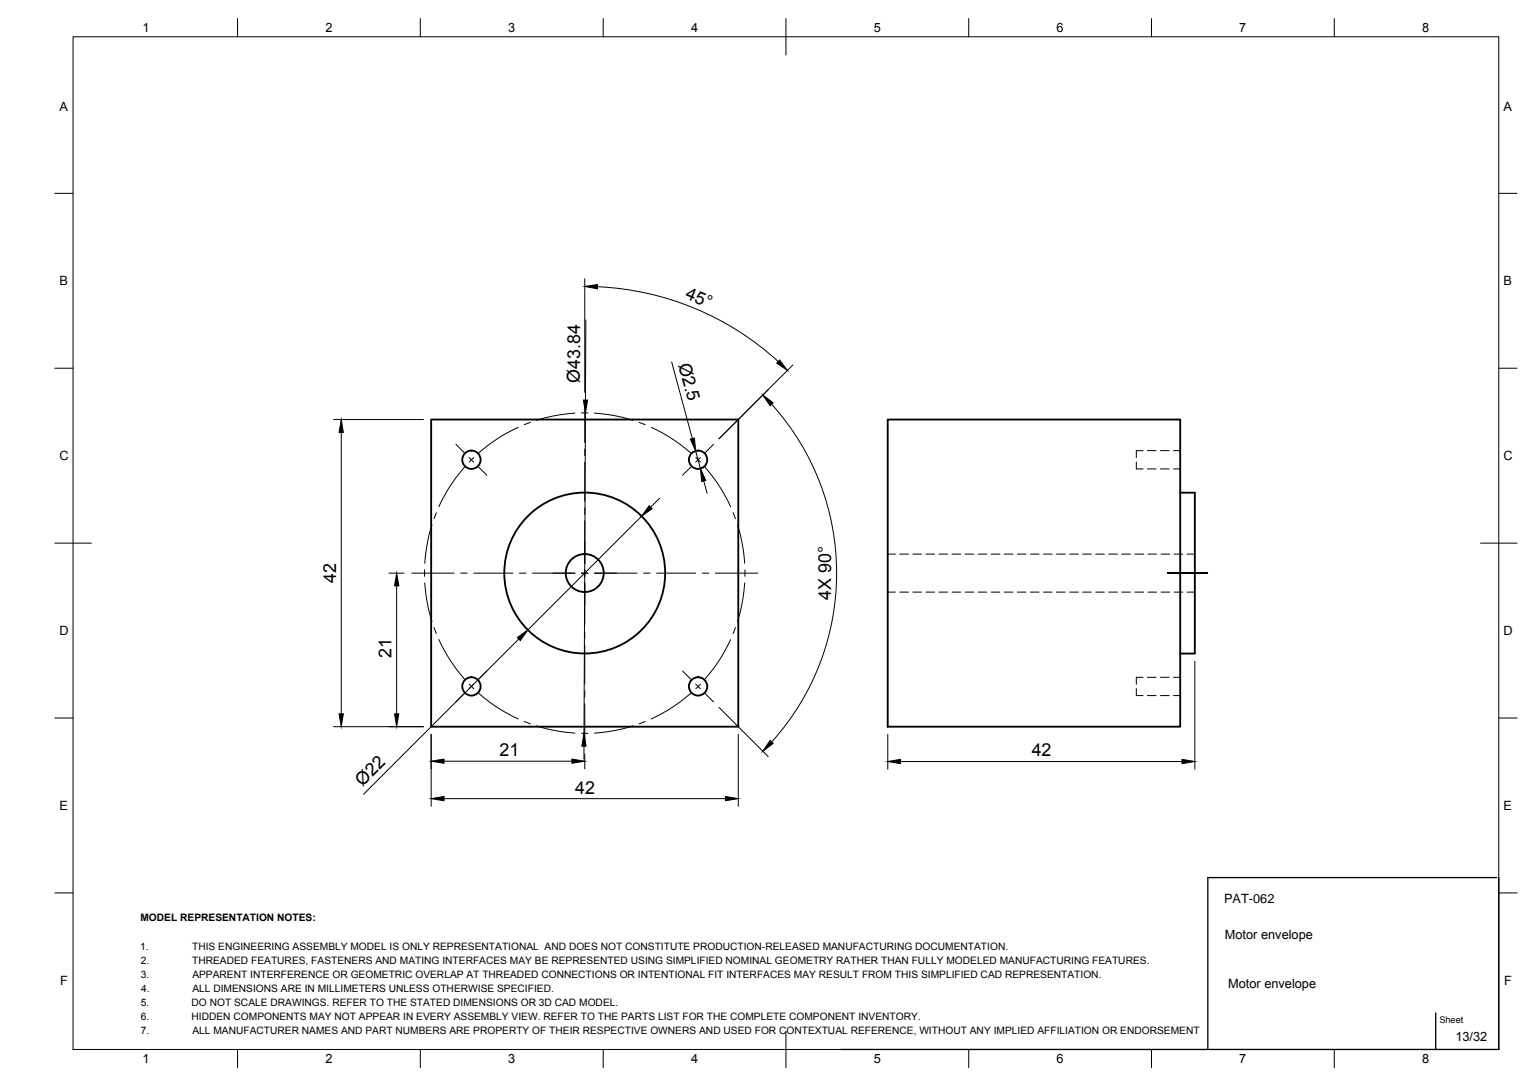
ISO-10303-21;
HEADER;
/* Generated by software containing ST-Developer
 * from STEP Tools, Inc. (www.steptools.com) 
 */

FILE_DESCRIPTION(
/* description */ ('Jaw-coupled motor to shaft test stand'),
/* implementation_level */ '2;1');

FILE_NAME(
/* name */ 'Motor envelope.step',
/* time_stamp */ '2026-10-27T10:46:06-07:00',
/* author */ (''),
/* organization */ (''),
/* preprocessor_version */ 'ST-DEVELOPER v20.2',
/* originating_system */ 'Autodesk Translation Framework v15.17.0.0',
/* authorisation */ '');

FILE_SCHEMA (('AUTOMOTIVE_DESIGN { 1 0 10303 214 3 1 1 }'));
ENDSEC;

DATA;
#10=MECHANICAL_DESIGN_GEOMETRIC_PRESENTATION_REPRESENTATION('',(#348),#19361);
#284=SHAPE_REPRESENTATION_RELATIONSHIP('SRR','None',#19498,#316);
#316=ADVANCED_BREP_SHAPE_REPRESENTATION('',(#381),#19334);
#348=STYLED_ITEM('',(#19739),#381);
#381=MANIFOLD_SOLID_BREP('Body1',#10992);
#437=FACE_BOUND('',#1741,.T.);
#438=FACE_BOUND('',#1744,.T.);
#439=FACE_BOUND('',#1745,.T.);
#440=FACE_BOUND('',#1746,.T.);
#441=FACE_BOUND('',#1747,.T.);
#442=FACE_BOUND('',#1748,.T.);
#443=FACE_BOUND('',#1751,.T.);
#550=PLANE('',#11484);
#551=PLANE('',#11488);
#552=PLANE('',#11492);
#553=PLANE('',#11496);
#554=PLANE('',#11500);
#555=PLANE('',#11504);
#556=PLANE('',#11505);
#557=PLANE('',#11506);
#558=PLANE('',#11507);
#559=PLANE('',#11508);
#560=PLANE('',#11509);
#1077=FACE_OUTER_BOUND('',#1731,.T.);
#1078=FACE_OUTER_BOUND('',#1732,.T.);
#1079=FACE_OUTER_BOUND('',#1733,.T.);
#1080=FACE_OUTER_BOUND('',#1734,.T.);
#1081=FACE_OUTER_BOUND('',#1735,.T.);
#1082=FACE_OUTER_BOUND('',#1736,.T.);
#1083=FACE_OUTER_BOUND('',#1737,.T.);
#1084=FACE_OUTER_BOUND('',#1738,.T.);
#1085=FACE_OUTER_BOUND('',#1739,.T.);
#1086=FACE_OUTER_BOUND('',#1740,.T.);
#1087=FACE_OUTER_BOUND('',#1742,.T.);
#1088=FACE_OUTER_BOUND('',#1743,.T.);
#1089=FACE_OUTER_BOUND('',#1749,.T.);
#1090=FACE_OUTER_BOUND('',#1750,.T.);
#1091=FACE_OUTER_BOUND('',#1752,.T.);
#1092=FACE_OUTER_BOUND('',#1753,.T.);
#1093=FACE_OUTER_BOUND('',#1754,.T.);
#1731=EDGE_LOOP('',(#7580,#7581,#7582,#7583));
#1732=EDGE_LOOP('',(#7584));
#1733=EDGE_LOOP('',(#7585,#7586,#7587,#7588));
#1734=EDGE_LOOP('',(#7589));
#1735=EDGE_LOOP('',(#7590,#7591,#7592,#7593));
#1736=EDGE_LOOP('',(#7594));
#1737=EDGE_LOOP('',(#7595,#7596,#7597,#7598));
#1738=EDGE_LOOP('',(#7599));
#1739=EDGE_LOOP('',(#7600,#7601,#7602,#7603));
#1740=EDGE_LOOP('',(#7604));
#1741=EDGE_LOOP('',(#7605));
#1742=EDGE_LOOP('',(#7606,#7607,#7608,#7609));
#1743=EDGE_LOOP('',(#7610,#7611,#7612,#7613));
#1744=EDGE_LOOP('',(#7614));
#1745=EDGE_LOOP('',(#7615));
#1746=EDGE_LOOP('',(#7616));
#1747=EDGE_LOOP('',(#7617));
#1748=EDGE_LOOP('',(#7618));
#1749=EDGE_LOOP('',(#7619,#7620,#7621,#7622));
#1750=EDGE_LOOP('',(#7623,#7624,#7625,#7626));
#1751=EDGE_LOOP('',(#7627));
#1752=EDGE_LOOP('',(#7628,#7629,#7630,#7631));
#1753=EDGE_LOOP('',(#7632,#7633,#7634,#7635));
#1754=EDGE_LOOP('',(#7636,#7637,#7638,#7639));
#2450=LINE('',#15692,#3603);
#2451=LINE('',#15699,#3604);
#2452=LINE('',#15706,#3605);
#2453=LINE('',#15713,#3606);
#2454=LINE('',#15720,#3607);
#2455=LINE('',#15728,#3608);
#2456=LINE('',#15732,#3609);
#2457=LINE('',#15734,#3610);
#2458=LINE('',#15736,#3611);
#2459=LINE('',#15737,#3612);
#2460=LINE('',#15740,#3613);
#2461=LINE('',#15742,#3614);
#2462=LINE('',#15743,#3615);
#2463=LINE('',#15746,#3616);
#2464=LINE('',#15748,#3617);
#2465=LINE('',#15749,#3618);
#2466=LINE('',#15751,#3619);
#2467=LINE('',#15752,#3620);
#3603=VECTOR('',#12635,0.125);
#3604=VECTOR('',#12644,0.125);
#3605=VECTOR('',#12653,0.125);
#3606=VECTOR('',#12662,0.125);
#3607=VECTOR('',#12671,1.1);
#3608=VECTOR('',#12682,0.26);
#3609=VECTOR('',#12685,1.);
#3610=VECTOR('',#12686,1.);
#3611=VECTOR('',#12687,1.);
#3612=VECTOR('',#12688,1.);
#3613=VECTOR('',#12691,1.);
#3614=VECTOR('',#12692,1.);
#3615=VECTOR('',#12693,1.);
#3616=VECTOR('',#12696,1.);
#3617=VECTOR('',#12697,1.);
#3618=VECTOR('',#12698,1.);
#3619=VECTOR('',#12701,1.);
#3620=VECTOR('',#12702,1.);
#4723=CIRCLE('',#11482,0.125);
#4724=CIRCLE('',#11483,0.125);
#4725=CIRCLE('',#11486,0.125);
#4726=CIRCLE('',#11487,0.125);
#4727=CIRCLE('',#11490,0.125);
#4728=CIRCLE('',#11491,0.125);
#4729=CIRCLE('',#11494,0.125);
#4730=CIRCLE('',#11495,0.125);
#4731=CIRCLE('',#11498,1.1);
#4732=CIRCLE('',#11499,1.1);
#4733=CIRCLE('',#11501,0.26);
#4734=CIRCLE('',#11503,0.26);
#5021=VERTEX_POINT('',#15689);
#5022=VERTEX_POINT('',#15691);
#5023=VERTEX_POINT('',#15696);
#5024=VERTEX_POINT('',#15698);
#5025=VERTEX_POINT('',#15703);
#5026=VERTEX_POINT('',#15705);
#5027=VERTEX_POINT('',#15710);
#5028=VERTEX_POINT('',#15712);
#5029=VERTEX_POINT('',#15717);
#5030=VERTEX_POINT('',#15719);
#5031=VERTEX_POINT('',#15723);
#5032=VERTEX_POINT('',#15726);
#5033=VERTEX_POINT('',#15730);
#5034=VERTEX_POINT('',#15731);
#5035=VERTEX_POINT('',#15733);
#5036=VERTEX_POINT('',#15735);
#5037=VERTEX_POINT('',#15739);
#5038=VERTEX_POINT('',#15741);
#5039=VERTEX_POINT('',#15745);
#5040=VERTEX_POINT('',#15747);
#6001=EDGE_CURVE('',#5021,#5021,#4723,.T.);
#6002=EDGE_CURVE('',#5021,#5022,#2450,.T.);
#6003=EDGE_CURVE('',#5022,#5022,#4724,.T.);
#6004=EDGE_CURVE('',#5023,#5023,#4725,.T.);
#6005=EDGE_CURVE('',#5023,#5024,#2451,.T.);
#6006=EDGE_CURVE('',#5024,#5024,#4726,.T.);
#6007=EDGE_CURVE('',#5025,#5025,#4727,.T.);
#6008=EDGE_CURVE('',#5025,#5026,#2452,.T.);
#6009=EDGE_CURVE('',#5026,#5026,#4728,.T.);
#6010=EDGE_CURVE('',#5027,#5027,#4729,.T.);
#6011=EDGE_CURVE('',#5027,#5028,#2453,.T.);
#6012=EDGE_CURVE('',#5028,#5028,#4730,.T.);
#6013=EDGE_CURVE('',#5029,#5029,#4731,.T.);
#6014=EDGE_CURVE('',#5029,#5030,#2454,.T.);
#6015=EDGE_CURVE('',#5030,#5030,#4732,.T.);
#6016=EDGE_CURVE('',#5031,#5031,#4733,.T.);
#6017=EDGE_CURVE('',#5032,#5032,#4734,.T.);
#6018=EDGE_CURVE('',#5032,#5031,#2455,.T.);
#6019=EDGE_CURVE('',#5033,#5034,#2456,.T.);
#6020=EDGE_CURVE('',#5034,#5035,#2457,.T.);
#6021=EDGE_CURVE('',#5036,#5035,#2458,.T.);
#6022=EDGE_CURVE('',#5033,#5036,#2459,.T.);
#6023=EDGE_CURVE('',#5037,#5033,#2460,.T.);
#6024=EDGE_CURVE('',#5038,#5036,#2461,.T.);
#6025=EDGE_CURVE('',#5037,#5038,#2462,.T.);
#6026=EDGE_CURVE('',#5039,#5037,#2463,.T.);
#6027=EDGE_CURVE('',#5040,#5038,#2464,.T.);
#6028=EDGE_CURVE('',#5039,#5040,#2465,.T.);
#6029=EDGE_CURVE('',#5034,#5039,#2466,.T.);
#6030=EDGE_CURVE('',#5035,#5040,#2467,.T.);
#7580=ORIENTED_EDGE('',*,*,#6001,.F.);
#7581=ORIENTED_EDGE('',*,*,#6002,.T.);
#7582=ORIENTED_EDGE('',*,*,#6003,.F.);
#7583=ORIENTED_EDGE('',*,*,#6002,.F.);
#7584=ORIENTED_EDGE('',*,*,#6001,.T.);
#7585=ORIENTED_EDGE('',*,*,#6004,.F.);
#7586=ORIENTED_EDGE('',*,*,#6005,.T.);
#7587=ORIENTED_EDGE('',*,*,#6006,.F.);
#7588=ORIENTED_EDGE('',*,*,#6005,.F.);
#7589=ORIENTED_EDGE('',*,*,#6004,.T.);
#7590=ORIENTED_EDGE('',*,*,#6007,.F.);
#7591=ORIENTED_EDGE('',*,*,#6008,.T.);
#7592=ORIENTED_EDGE('',*,*,#6009,.F.);
#7593=ORIENTED_EDGE('',*,*,#6008,.F.);
#7594=ORIENTED_EDGE('',*,*,#6007,.T.);
#7595=ORIENTED_EDGE('',*,*,#6010,.F.);
#7596=ORIENTED_EDGE('',*,*,#6011,.T.);
#7597=ORIENTED_EDGE('',*,*,#6012,.F.);
#7598=ORIENTED_EDGE('',*,*,#6011,.F.);
#7599=ORIENTED_EDGE('',*,*,#6010,.T.);
#7600=ORIENTED_EDGE('',*,*,#6013,.F.);
#7601=ORIENTED_EDGE('',*,*,#6014,.T.);
#7602=ORIENTED_EDGE('',*,*,#6015,.F.);
#7603=ORIENTED_EDGE('',*,*,#6014,.F.);
#7604=ORIENTED_EDGE('',*,*,#6013,.T.);
#7605=ORIENTED_EDGE('',*,*,#6016,.T.);
#7606=ORIENTED_EDGE('',*,*,#6017,.F.);
#7607=ORIENTED_EDGE('',*,*,#6018,.T.);
#7608=ORIENTED_EDGE('',*,*,#6016,.F.);
#7609=ORIENTED_EDGE('',*,*,#6018,.F.);
#7610=ORIENTED_EDGE('',*,*,#6019,.T.);
#7611=ORIENTED_EDGE('',*,*,#6020,.T.);
#7612=ORIENTED_EDGE('',*,*,#6021,.F.);
#7613=ORIENTED_EDGE('',*,*,#6022,.F.);
#7614=ORIENTED_EDGE('',*,*,#6015,.T.);
#7615=ORIENTED_EDGE('',*,*,#6012,.T.);
#7616=ORIENTED_EDGE('',*,*,#6009,.T.);
#7617=ORIENTED_EDGE('',*,*,#6006,.T.);
#7618=ORIENTED_EDGE('',*,*,#6003,.T.);
#7619=ORIENTED_EDGE('',*,*,#6023,.T.);
#7620=ORIENTED_EDGE('',*,*,#6022,.T.);
#7621=ORIENTED_EDGE('',*,*,#6024,.F.);
#7622=ORIENTED_EDGE('',*,*,#6025,.F.);
#7623=ORIENTED_EDGE('',*,*,#6026,.T.);
#7624=ORIENTED_EDGE('',*,*,#6025,.T.);
#7625=ORIENTED_EDGE('',*,*,#6027,.F.);
#7626=ORIENTED_EDGE('',*,*,#6028,.F.);
#7627=ORIENTED_EDGE('',*,*,#6017,.T.);
#7628=ORIENTED_EDGE('',*,*,#6029,.T.);
#7629=ORIENTED_EDGE('',*,*,#6028,.T.);
#7630=ORIENTED_EDGE('',*,*,#6030,.F.);
#7631=ORIENTED_EDGE('',*,*,#6020,.F.);
#7632=ORIENTED_EDGE('',*,*,#6030,.T.);
#7633=ORIENTED_EDGE('',*,*,#6027,.T.);
#7634=ORIENTED_EDGE('',*,*,#6024,.T.);
#7635=ORIENTED_EDGE('',*,*,#6021,.T.);
#7636=ORIENTED_EDGE('',*,*,#6029,.F.);
#7637=ORIENTED_EDGE('',*,*,#6019,.F.);
#7638=ORIENTED_EDGE('',*,*,#6023,.F.);
#7639=ORIENTED_EDGE('',*,*,#6026,.F.);
#10291=CYLINDRICAL_SURFACE('',#11481,0.125);
#10292=CYLINDRICAL_SURFACE('',#11485,0.125);
#10293=CYLINDRICAL_SURFACE('',#11489,0.125);
#10294=CYLINDRICAL_SURFACE('',#11493,0.125);
#10295=CYLINDRICAL_SURFACE('',#11497,1.1);
#10296=CYLINDRICAL_SURFACE('',#11502,0.26);
#10419=ADVANCED_FACE('',(#1077),#10291,.F.);
#10420=ADVANCED_FACE('',(#1078),#550,.T.);
#10421=ADVANCED_FACE('',(#1079),#10292,.F.);
#10422=ADVANCED_FACE('',(#1080),#551,.T.);
#10423=ADVANCED_FACE('',(#1081),#10293,.F.);
#10424=ADVANCED_FACE('',(#1082),#552,.T.);
#10425=ADVANCED_FACE('',(#1083),#10294,.F.);
#10426=ADVANCED_FACE('',(#1084),#553,.T.);
#10427=ADVANCED_FACE('',(#1085),#10295,.T.);
#10428=ADVANCED_FACE('',(#1086,#437),#554,.T.);
#10429=ADVANCED_FACE('',(#1087),#10296,.F.);
#10430=ADVANCED_FACE('',(#1088,#438,#439,#440,#441,#442),#555,.T.);
#10431=ADVANCED_FACE('',(#1089),#556,.T.);
#10432=ADVANCED_FACE('',(#1090,#443),#557,.T.);
#10433=ADVANCED_FACE('',(#1091),#558,.T.);
#10434=ADVANCED_FACE('',(#1092),#559,.T.);
#10435=ADVANCED_FACE('',(#1093),#560,.F.);
#10992=CLOSED_SHELL('',(#10419,#10420,#10421,#10422,#10423,#10424,#10425,
#10426,#10427,#10428,#10429,#10430,#10431,#10432,#10433,#10434,#10435));
#11480=AXIS2_PLACEMENT_3D('',#15687,#12629,#12630);
#11481=AXIS2_PLACEMENT_3D('',#15688,#12631,#12632);
#11482=AXIS2_PLACEMENT_3D('',#15690,#12633,#12634);
#11483=AXIS2_PLACEMENT_3D('',#15693,#12636,#12637);
#11484=AXIS2_PLACEMENT_3D('',#15694,#12638,#12639);
#11485=AXIS2_PLACEMENT_3D('',#15695,#12640,#12641);
#11486=AXIS2_PLACEMENT_3D('',#15697,#12642,#12643);
#11487=AXIS2_PLACEMENT_3D('',#15700,#12645,#12646);
#11488=AXIS2_PLACEMENT_3D('',#15701,#12647,#12648);
#11489=AXIS2_PLACEMENT_3D('',#15702,#12649,#12650);
#11490=AXIS2_PLACEMENT_3D('',#15704,#12651,#12652);
#11491=AXIS2_PLACEMENT_3D('',#15707,#12654,#12655);
#11492=AXIS2_PLACEMENT_3D('',#15708,#12656,#12657);
#11493=AXIS2_PLACEMENT_3D('',#15709,#12658,#12659);
#11494=AXIS2_PLACEMENT_3D('',#15711,#12660,#12661);
#11495=AXIS2_PLACEMENT_3D('',#15714,#12663,#12664);
#11496=AXIS2_PLACEMENT_3D('',#15715,#12665,#12666);
#11497=AXIS2_PLACEMENT_3D('',#15716,#12667,#12668);
#11498=AXIS2_PLACEMENT_3D('',#15718,#12669,#12670);
#11499=AXIS2_PLACEMENT_3D('',#15721,#12672,#12673);
#11500=AXIS2_PLACEMENT_3D('',#15722,#12674,#12675);
#11501=AXIS2_PLACEMENT_3D('',#15724,#12676,#12677);
#11502=AXIS2_PLACEMENT_3D('',#15725,#12678,#12679);
#11503=AXIS2_PLACEMENT_3D('',#15727,#12680,#12681);
#11504=AXIS2_PLACEMENT_3D('',#15729,#12683,#12684);
#11505=AXIS2_PLACEMENT_3D('',#15738,#12689,#12690);
#11506=AXIS2_PLACEMENT_3D('',#15744,#12694,#12695);
#11507=AXIS2_PLACEMENT_3D('',#15750,#12699,#12700);
#11508=AXIS2_PLACEMENT_3D('',#15753,#12703,#12704);
#11509=AXIS2_PLACEMENT_3D('',#15754,#12705,#12706);
#12629=DIRECTION('axis',(0.,0.,1.));
#12630=DIRECTION('refdir',(1.,0.,0.));
#12631=DIRECTION('center_axis',(0.,1.,0.));
#12632=DIRECTION('ref_axis',(1.,0.,0.));
#12633=DIRECTION('center_axis',(0.,1.,0.));
#12634=DIRECTION('ref_axis',(1.,0.,0.));
#12635=DIRECTION('',(0.,1.,0.));
#12636=DIRECTION('center_axis',(0.,-1.,0.));
#12637=DIRECTION('ref_axis',(1.,0.,0.));
#12638=DIRECTION('center_axis',(0.,1.,0.));
#12639=DIRECTION('ref_axis',(1.,0.,0.));
#12640=DIRECTION('center_axis',(0.,1.,0.));
#12641=DIRECTION('ref_axis',(1.,0.,0.));
#12642=DIRECTION('center_axis',(0.,1.,0.));
#12643=DIRECTION('ref_axis',(1.,0.,0.));
#12644=DIRECTION('',(0.,1.,0.));
#12645=DIRECTION('center_axis',(0.,-1.,0.));
#12646=DIRECTION('ref_axis',(1.,0.,0.));
#12647=DIRECTION('center_axis',(0.,1.,0.));
#12648=DIRECTION('ref_axis',(1.,0.,0.));
#12649=DIRECTION('center_axis',(0.,1.,0.));
#12650=DIRECTION('ref_axis',(1.,0.,0.));
#12651=DIRECTION('center_axis',(0.,1.,0.));
#12652=DIRECTION('ref_axis',(1.,0.,0.));
#12653=DIRECTION('',(0.,1.,0.));
#12654=DIRECTION('center_axis',(0.,-1.,0.));
#12655=DIRECTION('ref_axis',(1.,0.,0.));
#12656=DIRECTION('center_axis',(0.,1.,0.));
#12657=DIRECTION('ref_axis',(1.,0.,0.));
#12658=DIRECTION('center_axis',(0.,1.,0.));
#12659=DIRECTION('ref_axis',(1.,0.,0.));
#12660=DIRECTION('center_axis',(0.,1.,0.));
#12661=DIRECTION('ref_axis',(1.,0.,0.));
#12662=DIRECTION('',(0.,1.,0.));
#12663=DIRECTION('center_axis',(0.,-1.,0.));
#12664=DIRECTION('ref_axis',(1.,0.,0.));
#12665=DIRECTION('center_axis',(0.,1.,0.));
#12666=DIRECTION('ref_axis',(1.,0.,0.));
#12667=DIRECTION('center_axis',(0.,1.,0.));
#12668=DIRECTION('ref_axis',(1.,0.,0.));
#12669=DIRECTION('center_axis',(0.,1.,0.));
#12670=DIRECTION('ref_axis',(1.,0.,0.));
#12671=DIRECTION('',(0.,-1.,0.));
#12672=DIRECTION('center_axis',(0.,-1.,0.));
#12673=DIRECTION('ref_axis',(1.,0.,0.));
#12674=DIRECTION('center_axis',(0.,1.,0.));
#12675=DIRECTION('ref_axis',(1.,0.,0.));
#12676=DIRECTION('center_axis',(0.,-1.,0.));
#12677=DIRECTION('ref_axis',(1.,0.,0.));
#12678=DIRECTION('center_axis',(0.,1.,0.));
#12679=DIRECTION('ref_axis',(1.,0.,0.));
#12680=DIRECTION('center_axis',(0.,1.,0.));
#12681=DIRECTION('ref_axis',(1.,0.,0.));
#12682=DIRECTION('',(0.,1.,0.));
#12683=DIRECTION('center_axis',(0.,1.,0.));
#12684=DIRECTION('ref_axis',(-1.,0.,0.));
#12685=DIRECTION('',(-1.,0.,0.));
#12686=DIRECTION('',(0.,0.,1.));
#12687=DIRECTION('',(-1.,0.,0.));
#12688=DIRECTION('',(0.,0.,1.));
#12689=DIRECTION('center_axis',(1.,0.,0.));
#12690=DIRECTION('ref_axis',(0.,1.,0.));
#12691=DIRECTION('',(0.,1.,0.));
#12692=DIRECTION('',(0.,1.,0.));
#12693=DIRECTION('',(0.,0.,1.));
#12694=DIRECTION('center_axis',(0.,-1.,0.));
#12695=DIRECTION('ref_axis',(1.,0.,0.));
#12696=DIRECTION('',(1.,0.,0.));
#12697=DIRECTION('',(1.,0.,0.));
#12698=DIRECTION('',(0.,0.,1.));
#12699=DIRECTION('center_axis',(-1.,0.,0.));
#12700=DIRECTION('ref_axis',(0.,-1.,0.));
#12701=DIRECTION('',(0.,-1.,0.));
#12702=DIRECTION('',(0.,-1.,0.));
#12703=DIRECTION('center_axis',(0.,0.,1.));
#12704=DIRECTION('ref_axis',(1.,0.,0.));
#12705=DIRECTION('center_axis',(0.,0.,1.));
#12706=DIRECTION('ref_axis',(1.,0.,0.));
#15687=CARTESIAN_POINT('',(0.,0.,0.));
#15688=CARTESIAN_POINT('Origin',(1.55,-8.2,2.67));
#15689=CARTESIAN_POINT('',(1.425,-8.2,2.67));
#15690=CARTESIAN_POINT('Origin',(1.55,-8.2,2.67));
#15691=CARTESIAN_POINT('',(1.425,-7.6,2.67));
#15692=CARTESIAN_POINT('',(1.425,-8.2,2.67));
#15693=CARTESIAN_POINT('Origin',(1.55,-7.6,2.67));
#15694=CARTESIAN_POINT('Origin',(1.55,-8.2,2.67));
#15695=CARTESIAN_POINT('Origin',(-1.55,-8.2,5.77));
#15696=CARTESIAN_POINT('',(-1.675,-8.2,5.77));
#15697=CARTESIAN_POINT('Origin',(-1.55,-8.2,5.77));
#15698=CARTESIAN_POINT('',(-1.675,-7.6,5.77));
#15699=CARTESIAN_POINT('',(-1.675,-8.2,5.77));
#15700=CARTESIAN_POINT('Origin',(-1.55,-7.6,5.77));
#15701=CARTESIAN_POINT('Origin',(-1.55,-8.2,5.77));
#15702=CARTESIAN_POINT('Origin',(-1.55,-8.2,2.67));
#15703=CARTESIAN_POINT('',(-1.675,-8.2,2.67));
#15704=CARTESIAN_POINT('Origin',(-1.55,-8.2,2.67));
#15705=CARTESIAN_POINT('',(-1.675,-7.6,2.67));
#15706=CARTESIAN_POINT('',(-1.675,-8.2,2.67));
#15707=CARTESIAN_POINT('Origin',(-1.55,-7.6,2.67));
#15708=CARTESIAN_POINT('Origin',(-1.55,-8.2,2.67));
#15709=CARTESIAN_POINT('Origin',(1.55,-8.2,5.77));
#15710=CARTESIAN_POINT('',(1.425,-8.2,5.77));
#15711=CARTESIAN_POINT('Origin',(1.55,-8.2,5.77));
#15712=CARTESIAN_POINT('',(1.425,-7.6,5.77));
#15713=CARTESIAN_POINT('',(1.425,-8.2,5.77));
#15714=CARTESIAN_POINT('Origin',(1.55,-7.6,5.77));
#15715=CARTESIAN_POINT('Origin',(1.55,-8.2,5.77));
#15716=CARTESIAN_POINT('Origin',(0.,-7.6,4.22));
#15717=CARTESIAN_POINT('',(-1.1,-7.4,4.22));
#15718=CARTESIAN_POINT('Origin',(0.,-7.4,4.22));
#15719=CARTESIAN_POINT('',(-1.1,-7.6,4.22));
#15720=CARTESIAN_POINT('',(-1.1,-7.6,4.22));
#15721=CARTESIAN_POINT('Origin',(0.,-7.6,4.22));
#15722=CARTESIAN_POINT('Origin',(0.,-7.4,4.22));
#15723=CARTESIAN_POINT('',(-0.26,-7.4,4.22));
#15724=CARTESIAN_POINT('Origin',(0.,-7.4,4.22));
#15725=CARTESIAN_POINT('Origin',(0.,-11.7,4.22));
#15726=CARTESIAN_POINT('',(-0.26,-11.6,4.22));
#15727=CARTESIAN_POINT('Origin',(0.,-11.6,4.22));
#15728=CARTESIAN_POINT('',(-0.26,-11.7,4.22));
#15729=CARTESIAN_POINT('Origin',(2.1,-7.6,2.12));
#15730=CARTESIAN_POINT('',(2.1,-7.6,2.12));
#15731=CARTESIAN_POINT('',(-2.1,-7.6,2.12));
#15732=CARTESIAN_POINT('',(2.1,-7.6,2.12));
#15733=CARTESIAN_POINT('',(-2.1,-7.6,6.32));
#15734=CARTESIAN_POINT('',(-2.1,-7.6,2.12));
#15735=CARTESIAN_POINT('',(2.1,-7.6,6.32));
#15736=CARTESIAN_POINT('',(2.1,-7.6,6.32));
#15737=CARTESIAN_POINT('',(2.1,-7.6,2.12));
#15738=CARTESIAN_POINT('Origin',(2.1,-11.6,2.12));
#15739=CARTESIAN_POINT('',(2.1,-11.6,2.12));
#15740=CARTESIAN_POINT('',(2.1,-11.6,2.12));
#15741=CARTESIAN_POINT('',(2.1,-11.6,6.32));
#15742=CARTESIAN_POINT('',(2.1,-11.6,6.32));
#15743=CARTESIAN_POINT('',(2.1,-11.6,2.12));
#15744=CARTESIAN_POINT('Origin',(-2.1,-11.6,2.12));
#15745=CARTESIAN_POINT('',(-2.1,-11.6,2.12));
#15746=CARTESIAN_POINT('',(-2.1,-11.6,2.12));
#15747=CARTESIAN_POINT('',(-2.1,-11.6,6.32));
#15748=CARTESIAN_POINT('',(-2.1,-11.6,6.32));
#15749=CARTESIAN_POINT('',(-2.1,-11.6,2.12));
#15750=CARTESIAN_POINT('Origin',(-2.1,-7.6,2.12));
#15751=CARTESIAN_POINT('',(-2.1,-7.6,2.12));
#15752=CARTESIAN_POINT('',(-2.1,-7.6,6.32));
#15753=CARTESIAN_POINT('Origin',(0.,-9.6,6.32));
#15754=CARTESIAN_POINT('Origin',(0.,-9.6,2.12));
#19296=UNCERTAINTY_MEASURE_WITH_UNIT(LENGTH_MEASURE(0.001),#19362,
'DISTANCE_ACCURACY_VALUE',
'Maximum model space distance between geometric entities at asserted c
onnectivities');
#19323=UNCERTAINTY_MEASURE_WITH_UNIT(LENGTH_MEASURE(0.001),#19362,
'DISTANCE_ACCURACY_VALUE',
'Maximum model space distance between geometric entities at asserted c
onnectivities');
#19334=(
GEOMETRIC_REPRESENTATION_CONTEXT(3)
GLOBAL_UNCERTAINTY_ASSIGNED_CONTEXT((#19296))
GLOBAL_UNIT_ASSIGNED_CONTEXT((#19362,#19364,#19365))
REPRESENTATION_CONTEXT('','3D')
);
#19361=(
GEOMETRIC_REPRESENTATION_CONTEXT(3)
GLOBAL_UNCERTAINTY_ASSIGNED_CONTEXT((#19323))
GLOBAL_UNIT_ASSIGNED_CONTEXT((#19362,#19364,#19365))
REPRESENTATION_CONTEXT('','3D')
);
#19362=(
LENGTH_UNIT()
NAMED_UNIT(*)
SI_UNIT(.CENTI.,.METRE.)
);
#19364=(
NAMED_UNIT(*)
PLANE_ANGLE_UNIT()
SI_UNIT($,.RADIAN.)
);
#19365=(
NAMED_UNIT(*)
SI_UNIT($,.STERADIAN.)
SOLID_ANGLE_UNIT()
);
#19376=SHAPE_DEFINITION_REPRESENTATION(#19413,#19498);
#19413=PRODUCT_DEFINITION_SHAPE('',$,#19536);
#19498=SHAPE_REPRESENTATION('',(#11480),#19334);
#19525=PRODUCT_DEFINITION_CONTEXT('part definition',#19638,'design');
#19536=PRODUCT_DEFINITION('Motor envelope','Motor envelope',#19573,#19525);
#19573=PRODUCT_DEFINITION_FORMATION('',$,#19650);
#19638=APPLICATION_CONTEXT(
'Core Data for Automotive Mechanical Design Process');
#19639=PRODUCT_CONTEXT('part definition',#19638,'mechanical');
#19650=PRODUCT('Motor envelope','Motor envelope','Motor envelope',(#19639));
#19733=COLOUR_RGB('Sky Blue',0.24,0.69,0.87);
#19734=FILL_AREA_STYLE_COLOUR('',#19733);
#19735=FILL_AREA_STYLE('',(#19734));
#19736=SURFACE_STYLE_FILL_AREA(#19735);
#19737=SURFACE_SIDE_STYLE('',(#19736));
#19738=SURFACE_STYLE_USAGE(.BOTH.,#19737);
#19739=PRESENTATION_STYLE_ASSIGNMENT((#19738));
ENDSEC;
END-ISO-10303-21;
